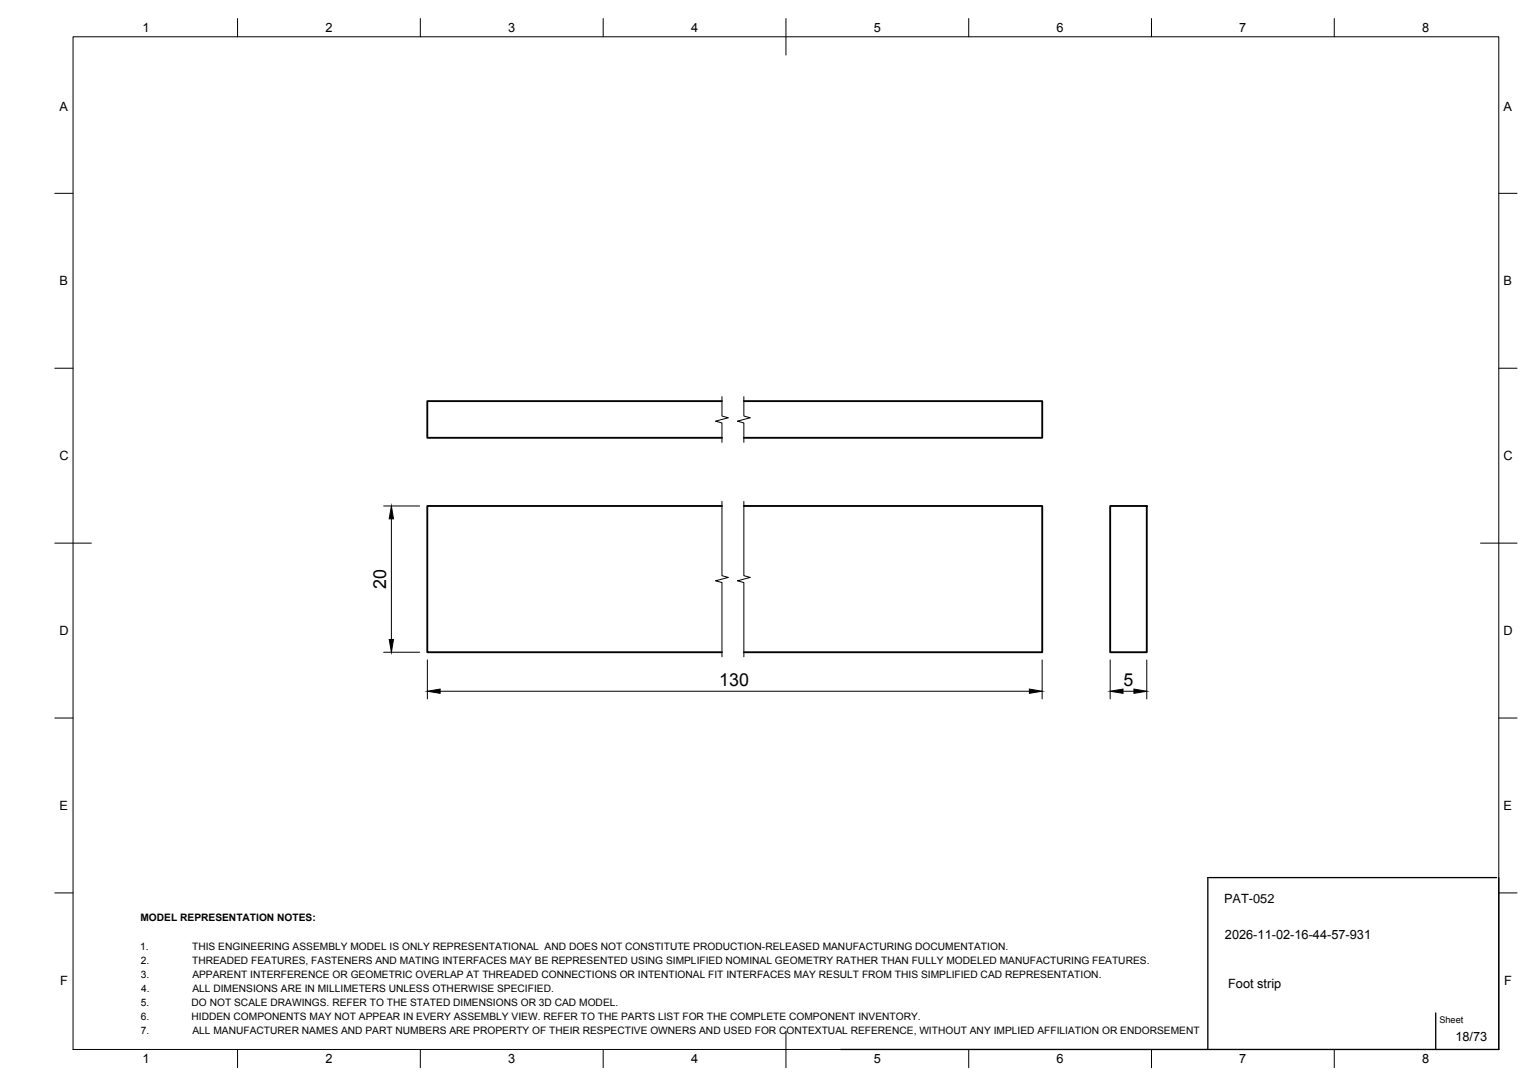
ISO-10303-21;
HEADER;
/* Generated by software containing ST-Developer
 * from STEP Tools, Inc. (www.steptools.com) 
 */

FILE_DESCRIPTION(
/* description */ ('Hand-crank gear train demonstrator'),
/* implementation_level */ '2;1');

FILE_NAME(
/* name */ 'Foot strip.step',
/* time_stamp */ '2026-10-28T03:22:13-07:00',
/* author */ (''),
/* organization */ (''),
/* preprocessor_version */ 'ST-DEVELOPER v20.2',
/* originating_system */ 'Autodesk Translation Framework v15.17.0.0',
/* authorisation */ '');

FILE_SCHEMA (('AUTOMOTIVE_DESIGN { 1 0 10303 214 3 1 1 }'));
ENDSEC;

DATA;
#10=MECHANICAL_DESIGN_GEOMETRIC_PRESENTATION_REPRESENTATION('',(#1229),#62758);
#1086=SHAPE_REPRESENTATION_RELATIONSHIP('SRR','None',#63060,#1150);
#1150=ADVANCED_BREP_SHAPE_REPRESENTATION('',(#1306),#62714);
#1229=STYLED_ITEM('',(#63448),#1306);
#1306=MANIFOLD_SOLID_BREP('Body1',#16411);
#1859=PLANE('',#17931);
#1860=PLANE('',#17932);
#1861=PLANE('',#17933);
#1862=PLANE('',#17934);
#1863=PLANE('',#17935);
#1864=PLANE('',#17936);
#2517=FACE_OUTER_BOUND('',#3651,.T.);
#2518=FACE_OUTER_BOUND('',#3652,.T.);
#2519=FACE_OUTER_BOUND('',#3653,.T.);
#2520=FACE_OUTER_BOUND('',#3654,.T.);
#2521=FACE_OUTER_BOUND('',#3655,.T.);
#2522=FACE_OUTER_BOUND('',#3656,.T.);
#3651=EDGE_LOOP('',(#12595,#12596,#12597,#12598));
#3652=EDGE_LOOP('',(#12599,#12600,#12601,#12602));
#3653=EDGE_LOOP('',(#12603,#12604,#12605,#12606));
#3654=EDGE_LOOP('',(#12607,#12608,#12609,#12610));
#3655=EDGE_LOOP('',(#12611,#12612,#12613,#12614));
#3656=EDGE_LOOP('',(#12615,#12616,#12617,#12618));
#4795=LINE('',#25860,#5927);
#4796=LINE('',#25862,#5928);
#4797=LINE('',#25864,#5929);
#4798=LINE('',#25865,#5930);
#4799=LINE('',#25868,#5931);
#4800=LINE('',#25870,#5932);
#4801=LINE('',#25871,#5933);
#4802=LINE('',#25874,#5934);
#4803=LINE('',#25876,#5935);
#4804=LINE('',#25877,#5936);
#4805=LINE('',#25879,#5937);
#4806=LINE('',#25880,#5938);
#5927=VECTOR('',#20888,1.);
#5928=VECTOR('',#20889,1.);
#5929=VECTOR('',#20890,1.);
#5930=VECTOR('',#20891,1.);
#5931=VECTOR('',#20894,1.);
#5932=VECTOR('',#20895,1.);
#5933=VECTOR('',#20896,1.);
#5934=VECTOR('',#20899,1.);
#5935=VECTOR('',#20900,1.);
#5936=VECTOR('',#20901,1.);
#5937=VECTOR('',#20904,1.);
#5938=VECTOR('',#20905,1.);
#7814=VERTEX_POINT('',#25858);
#7815=VERTEX_POINT('',#25859);
#7816=VERTEX_POINT('',#25861);
#7817=VERTEX_POINT('',#25863);
#7818=VERTEX_POINT('',#25867);
#7819=VERTEX_POINT('',#25869);
#7820=VERTEX_POINT('',#25873);
#7821=VERTEX_POINT('',#25875);
#9549=EDGE_CURVE('',#7814,#7815,#4795,.T.);
#9550=EDGE_CURVE('',#7815,#7816,#4796,.T.);
#9551=EDGE_CURVE('',#7817,#7816,#4797,.T.);
#9552=EDGE_CURVE('',#7814,#7817,#4798,.T.);
#9553=EDGE_CURVE('',#7818,#7814,#4799,.T.);
#9554=EDGE_CURVE('',#7819,#7817,#4800,.T.);
#9555=EDGE_CURVE('',#7818,#7819,#4801,.T.);
#9556=EDGE_CURVE('',#7820,#7818,#4802,.T.);
#9557=EDGE_CURVE('',#7821,#7819,#4803,.T.);
#9558=EDGE_CURVE('',#7820,#7821,#4804,.T.);
#9559=EDGE_CURVE('',#7815,#7820,#4805,.T.);
#9560=EDGE_CURVE('',#7816,#7821,#4806,.T.);
#12595=ORIENTED_EDGE('',*,*,#9549,.T.);
#12596=ORIENTED_EDGE('',*,*,#9550,.T.);
#12597=ORIENTED_EDGE('',*,*,#9551,.F.);
#12598=ORIENTED_EDGE('',*,*,#9552,.F.);
#12599=ORIENTED_EDGE('',*,*,#9553,.T.);
#12600=ORIENTED_EDGE('',*,*,#9552,.T.);
#12601=ORIENTED_EDGE('',*,*,#9554,.F.);
#12602=ORIENTED_EDGE('',*,*,#9555,.F.);
#12603=ORIENTED_EDGE('',*,*,#9556,.T.);
#12604=ORIENTED_EDGE('',*,*,#9555,.T.);
#12605=ORIENTED_EDGE('',*,*,#9557,.F.);
#12606=ORIENTED_EDGE('',*,*,#9558,.F.);
#12607=ORIENTED_EDGE('',*,*,#9559,.T.);
#12608=ORIENTED_EDGE('',*,*,#9558,.T.);
#12609=ORIENTED_EDGE('',*,*,#9560,.F.);
#12610=ORIENTED_EDGE('',*,*,#9550,.F.);
#12611=ORIENTED_EDGE('',*,*,#9560,.T.);
#12612=ORIENTED_EDGE('',*,*,#9557,.T.);
#12613=ORIENTED_EDGE('',*,*,#9554,.T.);
#12614=ORIENTED_EDGE('',*,*,#9551,.T.);
#12615=ORIENTED_EDGE('',*,*,#9559,.F.);
#12616=ORIENTED_EDGE('',*,*,#9549,.F.);
#12617=ORIENTED_EDGE('',*,*,#9553,.F.);
#12618=ORIENTED_EDGE('',*,*,#9556,.F.);
#15827=ADVANCED_FACE('',(#2517),#1859,.T.);
#15828=ADVANCED_FACE('',(#2518),#1860,.T.);
#15829=ADVANCED_FACE('',(#2519),#1861,.T.);
#15830=ADVANCED_FACE('',(#2520),#1862,.T.);
#15831=ADVANCED_FACE('',(#2521),#1863,.T.);
#15832=ADVANCED_FACE('',(#2522),#1864,.F.);
#16411=CLOSED_SHELL('',(#15827,#15828,#15829,#15830,#15831,#15832));
#17930=AXIS2_PLACEMENT_3D('',#25856,#20884,#20885);
#17931=AXIS2_PLACEMENT_3D('',#25857,#20886,#20887);
#17932=AXIS2_PLACEMENT_3D('',#25866,#20892,#20893);
#17933=AXIS2_PLACEMENT_3D('',#25872,#20897,#20898);
#17934=AXIS2_PLACEMENT_3D('',#25878,#20902,#20903);
#17935=AXIS2_PLACEMENT_3D('',#25881,#20906,#20907);
#17936=AXIS2_PLACEMENT_3D('',#25882,#20908,#20909);
#20884=DIRECTION('axis',(0.,0.,1.));
#20885=DIRECTION('refdir',(1.,0.,0.));
#20886=DIRECTION('center_axis',(0.,1.,0.));
#20887=DIRECTION('ref_axis',(-1.,0.,0.));
#20888=DIRECTION('',(-1.,0.,0.));
#20889=DIRECTION('',(0.,0.,1.));
#20890=DIRECTION('',(-1.,0.,0.));
#20891=DIRECTION('',(0.,0.,1.));
#20892=DIRECTION('center_axis',(1.,0.,0.));
#20893=DIRECTION('ref_axis',(0.,1.,0.));
#20894=DIRECTION('',(0.,1.,0.));
#20895=DIRECTION('',(0.,1.,0.));
#20896=DIRECTION('',(0.,0.,1.));
#20897=DIRECTION('center_axis',(0.,-1.,0.));
#20898=DIRECTION('ref_axis',(1.,0.,0.));
#20899=DIRECTION('',(1.,0.,0.));
#20900=DIRECTION('',(1.,0.,0.));
#20901=DIRECTION('',(0.,0.,1.));
#20902=DIRECTION('center_axis',(-1.,0.,0.));
#20903=DIRECTION('ref_axis',(0.,-1.,0.));
#20904=DIRECTION('',(0.,-1.,0.));
#20905=DIRECTION('',(0.,-1.,0.));
#20906=DIRECTION('center_axis',(0.,0.,1.));
#20907=DIRECTION('ref_axis',(1.,0.,0.));
#20908=DIRECTION('center_axis',(0.,0.,1.));
#20909=DIRECTION('ref_axis',(1.,0.,0.));
#25856=CARTESIAN_POINT('',(0.,0.,0.));
#25857=CARTESIAN_POINT('Origin',(-2.,6.5,-0.5));
#25858=CARTESIAN_POINT('',(-2.,6.5,-0.5));
#25859=CARTESIAN_POINT('',(-4.,6.5,-0.5));
#25860=CARTESIAN_POINT('',(-2.,6.5,-0.5));
#25861=CARTESIAN_POINT('',(-4.,6.5,0.));
#25862=CARTESIAN_POINT('',(-4.,6.5,-0.5));
#25863=CARTESIAN_POINT('',(-2.,6.5,0.));
#25864=CARTESIAN_POINT('',(-2.,6.5,0.));
#25865=CARTESIAN_POINT('',(-2.,6.5,-0.5));
#25866=CARTESIAN_POINT('Origin',(-2.,-6.5,-0.5));
#25867=CARTESIAN_POINT('',(-2.,-6.5,-0.5));
#25868=CARTESIAN_POINT('',(-2.,-6.5,-0.5));
#25869=CARTESIAN_POINT('',(-2.,-6.5,0.));
#25870=CARTESIAN_POINT('',(-2.,-6.5,0.));
#25871=CARTESIAN_POINT('',(-2.,-6.5,-0.5));
#25872=CARTESIAN_POINT('Origin',(-4.,-6.5,-0.5));
#25873=CARTESIAN_POINT('',(-4.,-6.5,-0.5));
#25874=CARTESIAN_POINT('',(-4.,-6.5,-0.5));
#25875=CARTESIAN_POINT('',(-4.,-6.5,0.));
#25876=CARTESIAN_POINT('',(-4.,-6.5,0.));
#25877=CARTESIAN_POINT('',(-4.,-6.5,-0.5));
#25878=CARTESIAN_POINT('Origin',(-4.,6.5,-0.5));
#25879=CARTESIAN_POINT('',(-4.,6.5,-0.5));
#25880=CARTESIAN_POINT('',(-4.,6.5,0.));
#25881=CARTESIAN_POINT('Origin',(-3.,0.,0.));
#25882=CARTESIAN_POINT('Origin',(-3.,0.,-0.5));
#62640=UNCERTAINTY_MEASURE_WITH_UNIT(LENGTH_MEASURE(0.001),#62759,
'DISTANCE_ACCURACY_VALUE',
'Maximum model space distance between geometric entities at asserted c
onnectivities');
#62684=UNCERTAINTY_MEASURE_WITH_UNIT(LENGTH_MEASURE(0.001),#62759,
'DISTANCE_ACCURACY_VALUE',
'Maximum model space distance between geometric entities at asserted c
onnectivities');
#62714=(
GEOMETRIC_REPRESENTATION_CONTEXT(3)
GLOBAL_UNCERTAINTY_ASSIGNED_CONTEXT((#62640))
GLOBAL_UNIT_ASSIGNED_CONTEXT((#62759,#62761,#62762))
REPRESENTATION_CONTEXT('','3D')
);
#62758=(
GEOMETRIC_REPRESENTATION_CONTEXT(3)
GLOBAL_UNCERTAINTY_ASSIGNED_CONTEXT((#62684))
GLOBAL_UNIT_ASSIGNED_CONTEXT((#62759,#62761,#62762))
REPRESENTATION_CONTEXT('','3D')
);
#62759=(
LENGTH_UNIT()
NAMED_UNIT(*)
SI_UNIT(.CENTI.,.METRE.)
);
#62761=(
NAMED_UNIT(*)
PLANE_ANGLE_UNIT()
SI_UNIT($,.RADIAN.)
);
#62762=(
NAMED_UNIT(*)
SI_UNIT($,.STERADIAN.)
SOLID_ANGLE_UNIT()
);
#62792=SHAPE_DEFINITION_REPRESENTATION(#62875,#63060);
#62875=PRODUCT_DEFINITION_SHAPE('',$,#63134);
#63060=SHAPE_REPRESENTATION('',(#17930),#62714);
#63104=PRODUCT_DEFINITION_CONTEXT('part definition',#63325,'design');
#63134=PRODUCT_DEFINITION('Foot strip','Foot strip',#63207,#63104);
#63207=PRODUCT_DEFINITION_FORMATION('',$,#63356);
#63325=APPLICATION_CONTEXT(
'Core Data for Automotive Mechanical Design Process');
#63326=PRODUCT_CONTEXT('part definition',#63325,'mechanical');
#63356=PRODUCT('Foot strip','Foot strip','Foot strip',(#63326));
#63442=COLOUR_RGB('Light Blue',0.38,0.62,0.78);
#63443=FILL_AREA_STYLE_COLOUR('',#63442);
#63444=FILL_AREA_STYLE('',(#63443));
#63445=SURFACE_STYLE_FILL_AREA(#63444);
#63446=SURFACE_SIDE_STYLE('',(#63445));
#63447=SURFACE_STYLE_USAGE(.BOTH.,#63446);
#63448=PRESENTATION_STYLE_ASSIGNMENT((#63447));
ENDSEC;
END-ISO-10303-21;
